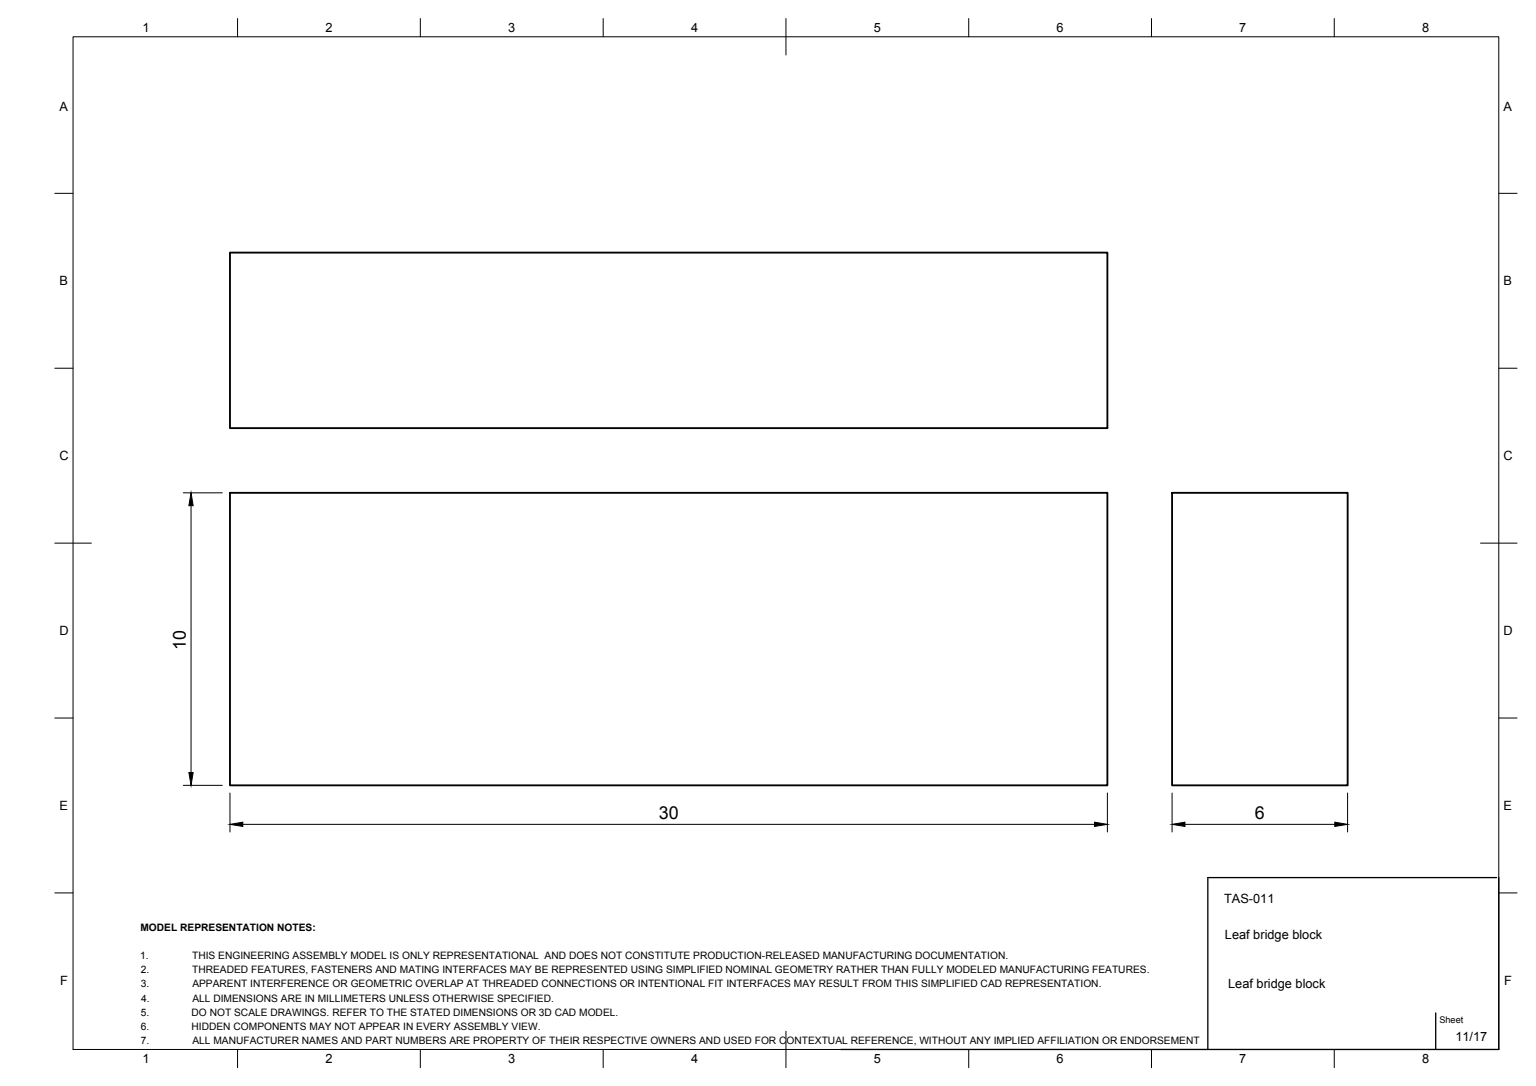
ISO-10303-21;
HEADER;
/* Generated by software containing ST-Developer
 * from STEP Tools, Inc. (www.steptools.com) 
 */

FILE_DESCRIPTION(
/* description */ (
'Independent manual bench leaf bending machine,200mm work width. Fabri
cated welded frame and folding leaf, repeated bushed and fully retaine
d hinge hardware, two handles with bonded grips, beveled clamping beam
 and modeledM12 clamp screws.2mm omitted-workpiece assembly reference 
gap, not a capacity claim. Native135deg hinge travel. Weld sizing, pro
duction fits, material condition, bending capacity, strength and life 
unassigned.'),
/* implementation_level */ '2;1');

FILE_NAME(
/* name */ 'Leaf bridge block.step',
/* time_stamp */ '2026-11-14T09:11:34-08:00',
/* author */ (''),
/* organization */ (''),
/* preprocessor_version */ 'ST-DEVELOPER v20.2',
/* originating_system */ 'Autodesk Translation Framework v15.17.0.0',
/* authorisation */ '');

FILE_SCHEMA (('AUTOMOTIVE_DESIGN { 1 0 10303 214 3 1 1 }'));
ENDSEC;

DATA;
#10=MECHANICAL_DESIGN_GEOMETRIC_PRESENTATION_REPRESENTATION('',(#456),#37701);
#420=SHAPE_REPRESENTATION_RELATIONSHIP('SRR','None',#37789,#438);
#438=ADVANCED_BREP_SHAPE_REPRESENTATION('',(#474),#37693);
#456=STYLED_ITEM('',(#37881),#474);
#474=MANIFOLD_SOLID_BREP('Body1',#4154);
#572=PLANE('',#4597);
#573=PLANE('',#4598);
#574=PLANE('',#4599);
#575=PLANE('',#4600);
#576=PLANE('',#4601);
#577=PLANE('',#4602);
#771=FACE_OUTER_BOUND('',#1009,.T.);
#772=FACE_OUTER_BOUND('',#1010,.T.);
#773=FACE_OUTER_BOUND('',#1011,.T.);
#774=FACE_OUTER_BOUND('',#1012,.T.);
#775=FACE_OUTER_BOUND('',#1013,.T.);
#776=FACE_OUTER_BOUND('',#1014,.T.);
#1009=EDGE_LOOP('',(#3673,#3674,#3675,#3676));
#1010=EDGE_LOOP('',(#3677,#3678,#3679,#3680));
#1011=EDGE_LOOP('',(#3681,#3682,#3683,#3684));
#1012=EDGE_LOOP('',(#3685,#3686,#3687,#3688));
#1013=EDGE_LOOP('',(#3689,#3690,#3691,#3692));
#1014=EDGE_LOOP('',(#3693,#3694,#3695,#3696));
#1266=LINE('',#37466,#1515);
#1267=LINE('',#37468,#1516);
#1268=LINE('',#37470,#1517);
#1269=LINE('',#37471,#1518);
#1270=LINE('',#37474,#1519);
#1271=LINE('',#37476,#1520);
#1272=LINE('',#37477,#1521);
#1273=LINE('',#37480,#1522);
#1274=LINE('',#37482,#1523);
#1275=LINE('',#37483,#1524);
#1276=LINE('',#37485,#1525);
#1277=LINE('',#37486,#1526);
#1515=VECTOR('',#5387,10.);
#1516=VECTOR('',#5388,10.);
#1517=VECTOR('',#5389,10.);
#1518=VECTOR('',#5390,10.);
#1519=VECTOR('',#5393,10.);
#1520=VECTOR('',#5394,10.);
#1521=VECTOR('',#5395,10.);
#1522=VECTOR('',#5398,10.);
#1523=VECTOR('',#5399,10.);
#1524=VECTOR('',#5400,10.);
#1525=VECTOR('',#5403,10.);
#1526=VECTOR('',#5404,10.);
#2007=VERTEX_POINT('',#37464);
#2008=VERTEX_POINT('',#37465);
#2009=VERTEX_POINT('',#37467);
#2010=VERTEX_POINT('',#37469);
#2011=VERTEX_POINT('',#37473);
#2012=VERTEX_POINT('',#37475);
#2013=VERTEX_POINT('',#37479);
#2014=VERTEX_POINT('',#37481);
#2570=EDGE_CURVE('',#2007,#2008,#1266,.T.);
#2571=EDGE_CURVE('',#2008,#2009,#1267,.T.);
#2572=EDGE_CURVE('',#2010,#2009,#1268,.T.);
#2573=EDGE_CURVE('',#2007,#2010,#1269,.T.);
#2574=EDGE_CURVE('',#2011,#2007,#1270,.T.);
#2575=EDGE_CURVE('',#2012,#2010,#1271,.T.);
#2576=EDGE_CURVE('',#2011,#2012,#1272,.T.);
#2577=EDGE_CURVE('',#2013,#2011,#1273,.T.);
#2578=EDGE_CURVE('',#2014,#2012,#1274,.T.);
#2579=EDGE_CURVE('',#2013,#2014,#1275,.T.);
#2580=EDGE_CURVE('',#2008,#2013,#1276,.T.);
#2581=EDGE_CURVE('',#2009,#2014,#1277,.T.);
#3673=ORIENTED_EDGE('',*,*,#2570,.T.);
#3674=ORIENTED_EDGE('',*,*,#2571,.T.);
#3675=ORIENTED_EDGE('',*,*,#2572,.F.);
#3676=ORIENTED_EDGE('',*,*,#2573,.F.);
#3677=ORIENTED_EDGE('',*,*,#2574,.T.);
#3678=ORIENTED_EDGE('',*,*,#2573,.T.);
#3679=ORIENTED_EDGE('',*,*,#2575,.F.);
#3680=ORIENTED_EDGE('',*,*,#2576,.F.);
#3681=ORIENTED_EDGE('',*,*,#2577,.T.);
#3682=ORIENTED_EDGE('',*,*,#2576,.T.);
#3683=ORIENTED_EDGE('',*,*,#2578,.F.);
#3684=ORIENTED_EDGE('',*,*,#2579,.F.);
#3685=ORIENTED_EDGE('',*,*,#2580,.T.);
#3686=ORIENTED_EDGE('',*,*,#2579,.T.);
#3687=ORIENTED_EDGE('',*,*,#2581,.F.);
#3688=ORIENTED_EDGE('',*,*,#2571,.F.);
#3689=ORIENTED_EDGE('',*,*,#2581,.T.);
#3690=ORIENTED_EDGE('',*,*,#2578,.T.);
#3691=ORIENTED_EDGE('',*,*,#2575,.T.);
#3692=ORIENTED_EDGE('',*,*,#2572,.T.);
#3693=ORIENTED_EDGE('',*,*,#2580,.F.);
#3694=ORIENTED_EDGE('',*,*,#2570,.F.);
#3695=ORIENTED_EDGE('',*,*,#2574,.F.);
#3696=ORIENTED_EDGE('',*,*,#2577,.F.);
#4101=ADVANCED_FACE('',(#771),#572,.T.);
#4102=ADVANCED_FACE('',(#772),#573,.T.);
#4103=ADVANCED_FACE('',(#773),#574,.T.);
#4104=ADVANCED_FACE('',(#774),#575,.T.);
#4105=ADVANCED_FACE('',(#775),#576,.T.);
#4106=ADVANCED_FACE('',(#776),#577,.F.);
#4154=CLOSED_SHELL('',(#4101,#4102,#4103,#4104,#4105,#4106));
#4596=AXIS2_PLACEMENT_3D('',#37462,#5383,#5384);
#4597=AXIS2_PLACEMENT_3D('',#37463,#5385,#5386);
#4598=AXIS2_PLACEMENT_3D('',#37472,#5391,#5392);
#4599=AXIS2_PLACEMENT_3D('',#37478,#5396,#5397);
#4600=AXIS2_PLACEMENT_3D('',#37484,#5401,#5402);
#4601=AXIS2_PLACEMENT_3D('',#37487,#5405,#5406);
#4602=AXIS2_PLACEMENT_3D('',#37488,#5407,#5408);
#5383=DIRECTION('axis',(0.,0.,1.));
#5384=DIRECTION('refdir',(1.,0.,0.));
#5385=DIRECTION('center_axis',(0.,1.,0.));
#5386=DIRECTION('ref_axis',(-1.,0.,0.));
#5387=DIRECTION('',(-1.,0.,0.));
#5388=DIRECTION('',(0.,0.,1.));
#5389=DIRECTION('',(-1.,0.,0.));
#5390=DIRECTION('',(0.,0.,1.));
#5391=DIRECTION('center_axis',(1.,0.,0.));
#5392=DIRECTION('ref_axis',(0.,1.,0.));
#5393=DIRECTION('',(0.,1.,0.));
#5394=DIRECTION('',(0.,1.,0.));
#5395=DIRECTION('',(0.,0.,1.));
#5396=DIRECTION('center_axis',(0.,-1.,0.));
#5397=DIRECTION('ref_axis',(1.,0.,0.));
#5398=DIRECTION('',(1.,0.,0.));
#5399=DIRECTION('',(1.,0.,0.));
#5400=DIRECTION('',(0.,0.,1.));
#5401=DIRECTION('center_axis',(-1.,0.,0.));
#5402=DIRECTION('ref_axis',(0.,-1.,0.));
#5403=DIRECTION('',(0.,-1.,0.));
#5404=DIRECTION('',(0.,-1.,0.));
#5405=DIRECTION('center_axis',(0.,0.,1.));
#5406=DIRECTION('ref_axis',(1.,0.,0.));
#5407=DIRECTION('center_axis',(0.,0.,1.));
#5408=DIRECTION('ref_axis',(1.,0.,0.));
#37462=CARTESIAN_POINT('',(0.,0.,0.));
#37463=CARTESIAN_POINT('Origin',(60.,3.,30.));
#37464=CARTESIAN_POINT('',(60.,3.,30.));
#37465=CARTESIAN_POINT('',(30.,3.,30.));
#37466=CARTESIAN_POINT('',(60.,3.,30.));
#37467=CARTESIAN_POINT('',(30.,3.,40.));
#37468=CARTESIAN_POINT('',(30.,3.,30.));
#37469=CARTESIAN_POINT('',(60.,3.,40.));
#37470=CARTESIAN_POINT('',(60.,3.,40.));
#37471=CARTESIAN_POINT('',(60.,3.,30.));
#37472=CARTESIAN_POINT('Origin',(60.,-3.,30.));
#37473=CARTESIAN_POINT('',(60.,-3.,30.));
#37474=CARTESIAN_POINT('',(60.,-3.,30.));
#37475=CARTESIAN_POINT('',(60.,-3.,40.));
#37476=CARTESIAN_POINT('',(60.,-3.,40.));
#37477=CARTESIAN_POINT('',(60.,-3.,30.));
#37478=CARTESIAN_POINT('Origin',(30.,-3.,30.));
#37479=CARTESIAN_POINT('',(30.,-3.,30.));
#37480=CARTESIAN_POINT('',(30.,-3.,30.));
#37481=CARTESIAN_POINT('',(30.,-3.,40.));
#37482=CARTESIAN_POINT('',(30.,-3.,40.));
#37483=CARTESIAN_POINT('',(30.,-3.,30.));
#37484=CARTESIAN_POINT('Origin',(30.,3.,30.));
#37485=CARTESIAN_POINT('',(30.,3.,30.));
#37486=CARTESIAN_POINT('',(30.,3.,40.));
#37487=CARTESIAN_POINT('Origin',(45.,0.,40.));
#37488=CARTESIAN_POINT('Origin',(45.,0.,30.));
#37673=UNCERTAINTY_MEASURE_WITH_UNIT(LENGTH_MEASURE(0.01),#37702,
'DISTANCE_ACCURACY_VALUE',
'Maximum model space distance between geometric entities at asserted c
onnectivities');
#37681=UNCERTAINTY_MEASURE_WITH_UNIT(LENGTH_MEASURE(0.01),#37702,
'DISTANCE_ACCURACY_VALUE',
'Maximum model space distance between geometric entities at asserted c
onnectivities');
#37693=(
GEOMETRIC_REPRESENTATION_CONTEXT(3)
GLOBAL_UNCERTAINTY_ASSIGNED_CONTEXT((#37673))
GLOBAL_UNIT_ASSIGNED_CONTEXT((#37702,#37704,#37705))
REPRESENTATION_CONTEXT('','3D')
);
#37701=(
GEOMETRIC_REPRESENTATION_CONTEXT(3)
GLOBAL_UNCERTAINTY_ASSIGNED_CONTEXT((#37681))
GLOBAL_UNIT_ASSIGNED_CONTEXT((#37702,#37704,#37705))
REPRESENTATION_CONTEXT('','3D')
);
#37702=(
LENGTH_UNIT()
NAMED_UNIT(*)
SI_UNIT(.MILLI.,.METRE.)
);
#37704=(
NAMED_UNIT(*)
PLANE_ANGLE_UNIT()
SI_UNIT($,.RADIAN.)
);
#37705=(
NAMED_UNIT(*)
SI_UNIT($,.STERADIAN.)
SOLID_ANGLE_UNIT()
);
#37717=SHAPE_DEFINITION_REPRESENTATION(#37736,#37789);
#37736=PRODUCT_DEFINITION_SHAPE('',$,#37809);
#37789=SHAPE_REPRESENTATION('',(#4596),#37693);
#37797=PRODUCT_DEFINITION_CONTEXT('part definition',#37856,'design');
#37809=PRODUCT_DEFINITION('Leaf bridge block','Leaf bridge block',#37828,
#37797);
#37828=PRODUCT_DEFINITION_FORMATION('',$,#37869);
#37856=APPLICATION_CONTEXT(
'Core Data for Automotive Mechanical Design Process');
#37857=PRODUCT_CONTEXT('part definition',#37856,'mechanical');
#37869=PRODUCT('Leaf bridge block','Leaf bridge block',$,(#37857));
#37881=PRESENTATION_STYLE_ASSIGNMENT((#37889));
#37889=SURFACE_STYLE_USAGE(.BOTH.,#37897);
#37897=SURFACE_SIDE_STYLE('',(#37905));
#37905=SURFACE_STYLE_FILL_AREA(#37913);
#37913=FILL_AREA_STYLE('Opaque(81,175,227)',(#37921));
#37921=FILL_AREA_STYLE_COLOUR('Opaque(81,175,227)',#37929);
#37929=COLOUR_RGB('Opaque(81,175,227)',0.317647058823529,0.686274509803922,
0.890196078431372);
ENDSEC;
END-ISO-10303-21;
